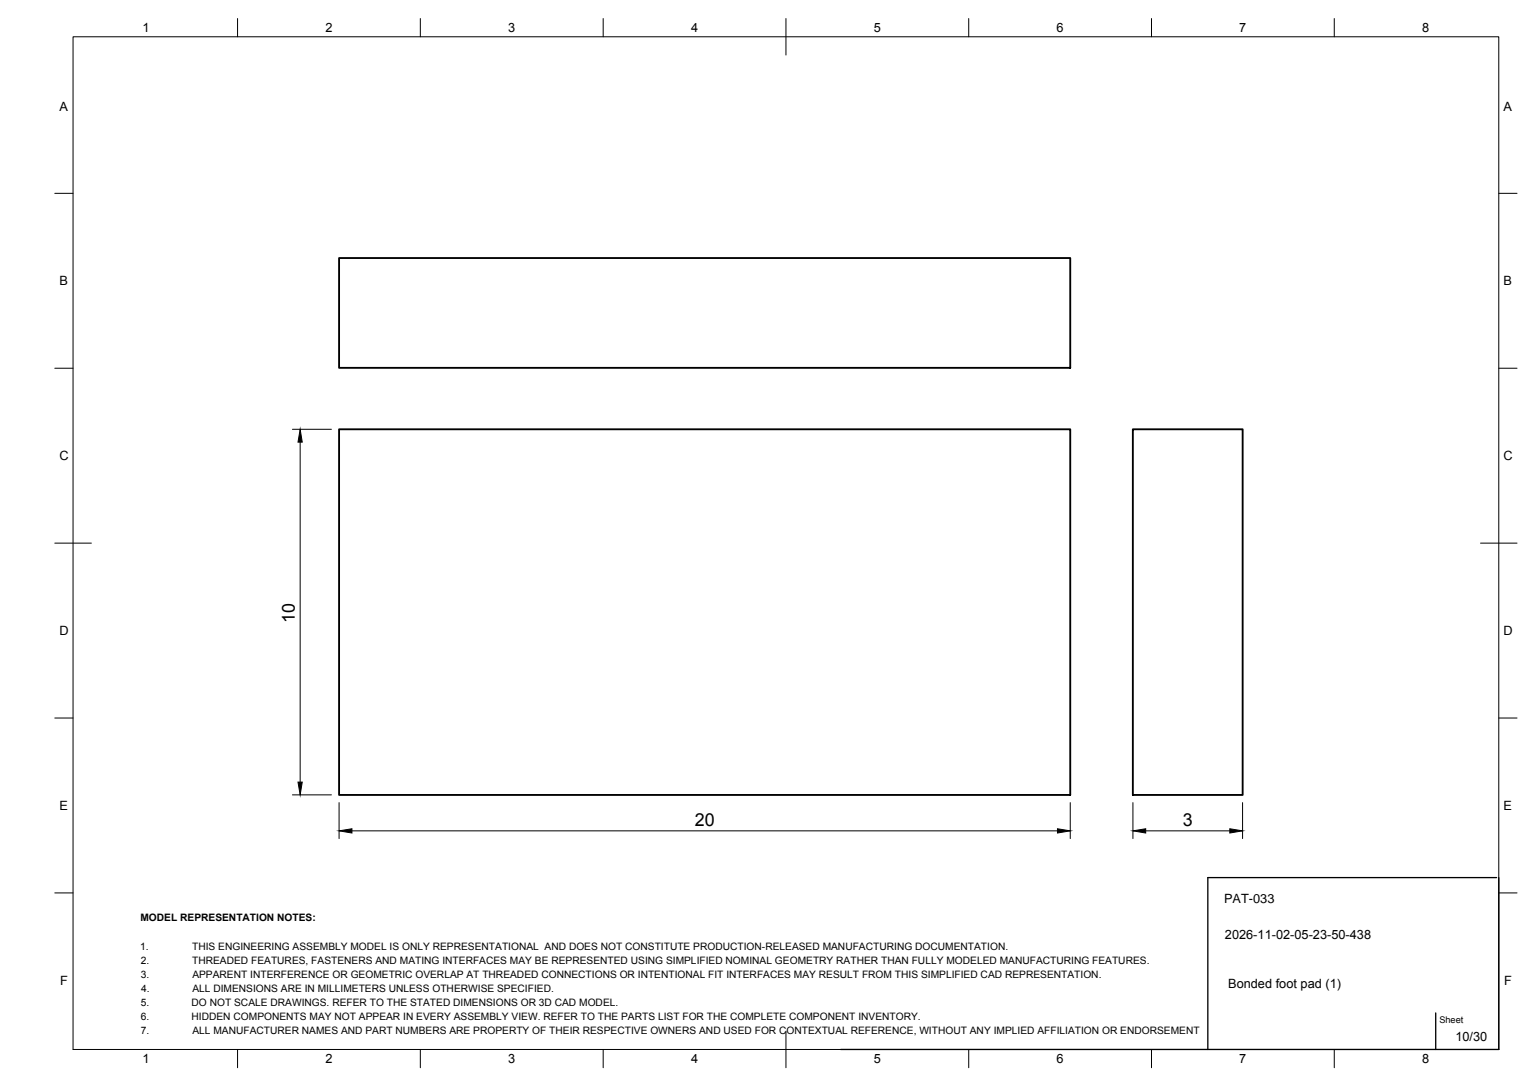
ISO-10303-21;
HEADER;
/* Generated by software containing ST-Developer
 * from STEP Tools, Inc. (www.steptools.com) 
 */

FILE_DESCRIPTION(
/* description */ ('Dual-rail gantry carriage'),
/* implementation_level */ '2;1');

FILE_NAME(
/* name */ 'Bonded foot pad (1).step',
/* time_stamp */ '2026-10-27T10:49:15-07:00',
/* author */ (''),
/* organization */ (''),
/* preprocessor_version */ 'ST-DEVELOPER v20.2',
/* originating_system */ 'Autodesk Translation Framework v15.17.0.0',
/* authorisation */ '');

FILE_SCHEMA (('AUTOMOTIVE_DESIGN { 1 0 10303 214 3 1 1 }'));
ENDSEC;

DATA;
#10=MECHANICAL_DESIGN_GEOMETRIC_PRESENTATION_REPRESENTATION('',(#590),#12804);
#528=SHAPE_REPRESENTATION_RELATIONSHIP('SRR','None',#13006,#559);
#559=ADVANCED_BREP_SHAPE_REPRESENTATION('',(#621),#12776);
#590=STYLED_ITEM('',(#13240),#621);
#621=MANIFOLD_SOLID_BREP('Body1',#7368);
#794=PLANE('',#7827);
#795=PLANE('',#7828);
#796=PLANE('',#7829);
#797=PLANE('',#7830);
#798=PLANE('',#7831);
#799=PLANE('',#7832);
#1094=FACE_OUTER_BOUND('',#1515,.T.);
#1095=FACE_OUTER_BOUND('',#1516,.T.);
#1096=FACE_OUTER_BOUND('',#1517,.T.);
#1097=FACE_OUTER_BOUND('',#1518,.T.);
#1098=FACE_OUTER_BOUND('',#1519,.T.);
#1099=FACE_OUTER_BOUND('',#1520,.T.);
#1515=EDGE_LOOP('',(#5283,#5284,#5285,#5286));
#1516=EDGE_LOOP('',(#5287,#5288,#5289,#5290));
#1517=EDGE_LOOP('',(#5291,#5292,#5293,#5294));
#1518=EDGE_LOOP('',(#5295,#5296,#5297,#5298));
#1519=EDGE_LOOP('',(#5299,#5300,#5301,#5302));
#1520=EDGE_LOOP('',(#5303,#5304,#5305,#5306));
#2024=LINE('',#10925,#2733);
#2025=LINE('',#10927,#2734);
#2026=LINE('',#10929,#2735);
#2027=LINE('',#10930,#2736);
#2028=LINE('',#10933,#2737);
#2029=LINE('',#10935,#2738);
#2030=LINE('',#10936,#2739);
#2031=LINE('',#10939,#2740);
#2032=LINE('',#10941,#2741);
#2033=LINE('',#10942,#2742);
#2034=LINE('',#10944,#2743);
#2035=LINE('',#10945,#2744);
#2733=VECTOR('',#8737,1.);
#2734=VECTOR('',#8738,1.);
#2735=VECTOR('',#8739,1.);
#2736=VECTOR('',#8740,1.);
#2737=VECTOR('',#8743,1.);
#2738=VECTOR('',#8744,1.);
#2739=VECTOR('',#8745,1.);
#2740=VECTOR('',#8748,1.);
#2741=VECTOR('',#8749,1.);
#2742=VECTOR('',#8750,1.);
#2743=VECTOR('',#8753,1.);
#2744=VECTOR('',#8754,1.);
#3638=VERTEX_POINT('',#10923);
#3639=VERTEX_POINT('',#10924);
#3640=VERTEX_POINT('',#10926);
#3641=VERTEX_POINT('',#10928);
#3642=VERTEX_POINT('',#10932);
#3643=VERTEX_POINT('',#10934);
#3644=VERTEX_POINT('',#10938);
#3645=VERTEX_POINT('',#10940);
#4264=EDGE_CURVE('',#3638,#3639,#2024,.T.);
#4265=EDGE_CURVE('',#3639,#3640,#2025,.T.);
#4266=EDGE_CURVE('',#3641,#3640,#2026,.T.);
#4267=EDGE_CURVE('',#3638,#3641,#2027,.T.);
#4268=EDGE_CURVE('',#3642,#3638,#2028,.T.);
#4269=EDGE_CURVE('',#3643,#3641,#2029,.T.);
#4270=EDGE_CURVE('',#3642,#3643,#2030,.T.);
#4271=EDGE_CURVE('',#3644,#3642,#2031,.T.);
#4272=EDGE_CURVE('',#3645,#3643,#2032,.T.);
#4273=EDGE_CURVE('',#3644,#3645,#2033,.T.);
#4274=EDGE_CURVE('',#3639,#3644,#2034,.T.);
#4275=EDGE_CURVE('',#3640,#3645,#2035,.T.);
#5283=ORIENTED_EDGE('',*,*,#4264,.T.);
#5284=ORIENTED_EDGE('',*,*,#4265,.T.);
#5285=ORIENTED_EDGE('',*,*,#4266,.F.);
#5286=ORIENTED_EDGE('',*,*,#4267,.F.);
#5287=ORIENTED_EDGE('',*,*,#4268,.T.);
#5288=ORIENTED_EDGE('',*,*,#4267,.T.);
#5289=ORIENTED_EDGE('',*,*,#4269,.F.);
#5290=ORIENTED_EDGE('',*,*,#4270,.F.);
#5291=ORIENTED_EDGE('',*,*,#4271,.T.);
#5292=ORIENTED_EDGE('',*,*,#4270,.T.);
#5293=ORIENTED_EDGE('',*,*,#4272,.F.);
#5294=ORIENTED_EDGE('',*,*,#4273,.F.);
#5295=ORIENTED_EDGE('',*,*,#4274,.T.);
#5296=ORIENTED_EDGE('',*,*,#4273,.T.);
#5297=ORIENTED_EDGE('',*,*,#4275,.F.);
#5298=ORIENTED_EDGE('',*,*,#4265,.F.);
#5299=ORIENTED_EDGE('',*,*,#4275,.T.);
#5300=ORIENTED_EDGE('',*,*,#4272,.T.);
#5301=ORIENTED_EDGE('',*,*,#4269,.T.);
#5302=ORIENTED_EDGE('',*,*,#4266,.T.);
#5303=ORIENTED_EDGE('',*,*,#4274,.F.);
#5304=ORIENTED_EDGE('',*,*,#4264,.F.);
#5305=ORIENTED_EDGE('',*,*,#4268,.F.);
#5306=ORIENTED_EDGE('',*,*,#4271,.F.);
#7020=ADVANCED_FACE('',(#1094),#794,.T.);
#7021=ADVANCED_FACE('',(#1095),#795,.T.);
#7022=ADVANCED_FACE('',(#1096),#796,.T.);
#7023=ADVANCED_FACE('',(#1097),#797,.T.);
#7024=ADVANCED_FACE('',(#1098),#798,.T.);
#7025=ADVANCED_FACE('',(#1099),#799,.F.);
#7368=CLOSED_SHELL('',(#7020,#7021,#7022,#7023,#7024,#7025));
#7826=AXIS2_PLACEMENT_3D('',#10921,#8733,#8734);
#7827=AXIS2_PLACEMENT_3D('',#10922,#8735,#8736);
#7828=AXIS2_PLACEMENT_3D('',#10931,#8741,#8742);
#7829=AXIS2_PLACEMENT_3D('',#10937,#8746,#8747);
#7830=AXIS2_PLACEMENT_3D('',#10943,#8751,#8752);
#7831=AXIS2_PLACEMENT_3D('',#10946,#8755,#8756);
#7832=AXIS2_PLACEMENT_3D('',#10947,#8757,#8758);
#8733=DIRECTION('axis',(0.,0.,1.));
#8734=DIRECTION('refdir',(1.,0.,0.));
#8735=DIRECTION('center_axis',(0.,1.,0.));
#8736=DIRECTION('ref_axis',(-1.,0.,0.));
#8737=DIRECTION('',(-1.,0.,0.));
#8738=DIRECTION('',(0.,0.,1.));
#8739=DIRECTION('',(-1.,0.,0.));
#8740=DIRECTION('',(0.,0.,1.));
#8741=DIRECTION('center_axis',(1.,0.,0.));
#8742=DIRECTION('ref_axis',(0.,1.,0.));
#8743=DIRECTION('',(0.,1.,0.));
#8744=DIRECTION('',(0.,1.,0.));
#8745=DIRECTION('',(0.,0.,1.));
#8746=DIRECTION('center_axis',(0.,-1.,0.));
#8747=DIRECTION('ref_axis',(1.,0.,0.));
#8748=DIRECTION('',(1.,0.,0.));
#8749=DIRECTION('',(1.,0.,0.));
#8750=DIRECTION('',(0.,0.,1.));
#8751=DIRECTION('center_axis',(-1.,0.,0.));
#8752=DIRECTION('ref_axis',(0.,-1.,0.));
#8753=DIRECTION('',(0.,-1.,0.));
#8754=DIRECTION('',(0.,-1.,0.));
#8755=DIRECTION('center_axis',(0.,0.,1.));
#8756=DIRECTION('ref_axis',(1.,0.,0.));
#8757=DIRECTION('center_axis',(0.,0.,1.));
#8758=DIRECTION('ref_axis',(1.,0.,0.));
#10921=CARTESIAN_POINT('',(0.,0.,0.));
#10922=CARTESIAN_POINT('Origin',(2.,12.5,-1.1));
#10923=CARTESIAN_POINT('',(2.,12.5,-1.1));
#10924=CARTESIAN_POINT('',(0.,12.5,-1.1));
#10925=CARTESIAN_POINT('',(2.,12.5,-1.1));
#10926=CARTESIAN_POINT('',(0.,12.5,-0.8));
#10927=CARTESIAN_POINT('',(0.,12.5,-1.1));
#10928=CARTESIAN_POINT('',(2.,12.5,-0.8));
#10929=CARTESIAN_POINT('',(2.,12.5,-0.8));
#10930=CARTESIAN_POINT('',(2.,12.5,-1.1));
#10931=CARTESIAN_POINT('Origin',(2.,11.5,-1.1));
#10932=CARTESIAN_POINT('',(2.,11.5,-1.1));
#10933=CARTESIAN_POINT('',(2.,11.5,-1.1));
#10934=CARTESIAN_POINT('',(2.,11.5,-0.8));
#10935=CARTESIAN_POINT('',(2.,11.5,-0.8));
#10936=CARTESIAN_POINT('',(2.,11.5,-1.1));
#10937=CARTESIAN_POINT('Origin',(0.,11.5,-1.1));
#10938=CARTESIAN_POINT('',(0.,11.5,-1.1));
#10939=CARTESIAN_POINT('',(0.,11.5,-1.1));
#10940=CARTESIAN_POINT('',(0.,11.5,-0.8));
#10941=CARTESIAN_POINT('',(0.,11.5,-0.8));
#10942=CARTESIAN_POINT('',(0.,11.5,-1.1));
#10943=CARTESIAN_POINT('Origin',(0.,12.5,-1.1));
#10944=CARTESIAN_POINT('',(0.,12.5,-1.1));
#10945=CARTESIAN_POINT('',(0.,12.5,-0.8));
#10946=CARTESIAN_POINT('Origin',(1.,12.,-0.8));
#10947=CARTESIAN_POINT('Origin',(1.,12.,-1.1));
#12740=UNCERTAINTY_MEASURE_WITH_UNIT(LENGTH_MEASURE(0.001),#12805,
'DISTANCE_ACCURACY_VALUE',
'Maximum model space distance between geometric entities at asserted c
onnectivities');
#12768=UNCERTAINTY_MEASURE_WITH_UNIT(LENGTH_MEASURE(0.001),#12805,
'DISTANCE_ACCURACY_VALUE',
'Maximum model space distance between geometric entities at asserted c
onnectivities');
#12776=(
GEOMETRIC_REPRESENTATION_CONTEXT(3)
GLOBAL_UNCERTAINTY_ASSIGNED_CONTEXT((#12740))
GLOBAL_UNIT_ASSIGNED_CONTEXT((#12805,#12807,#12808))
REPRESENTATION_CONTEXT('','3D')
);
#12804=(
GEOMETRIC_REPRESENTATION_CONTEXT(3)
GLOBAL_UNCERTAINTY_ASSIGNED_CONTEXT((#12768))
GLOBAL_UNIT_ASSIGNED_CONTEXT((#12805,#12807,#12808))
REPRESENTATION_CONTEXT('','3D')
);
#12805=(
LENGTH_UNIT()
NAMED_UNIT(*)
SI_UNIT(.CENTI.,.METRE.)
);
#12807=(
NAMED_UNIT(*)
PLANE_ANGLE_UNIT()
SI_UNIT($,.RADIAN.)
);
#12808=(
NAMED_UNIT(*)
SI_UNIT($,.STERADIAN.)
SOLID_ANGLE_UNIT()
);
#12816=SHAPE_DEFINITION_REPRESENTATION(#12851,#13006);
#12851=PRODUCT_DEFINITION_SHAPE('',$,#13042);
#13006=SHAPE_REPRESENTATION('',(#7826),#12776);
#13034=PRODUCT_DEFINITION_CONTEXT('part definition',#13141,'design');
#13042=PRODUCT_DEFINITION('Bonded foot pad (1)','Bonded foot pad (1)',#13077,
#13034);
#13077=PRODUCT_DEFINITION_FORMATION('',$,#13150);
#13141=APPLICATION_CONTEXT(
'Core Data for Automotive Mechanical Design Process');
#13142=PRODUCT_CONTEXT('part definition',#13141,'mechanical');
#13150=PRODUCT('Bonded foot pad (1)','Bonded foot pad (1)',
'Bonded foot pad (1)',(#13142));
#13234=COLOUR_RGB('Sky Blue',0.24,0.69,0.87);
#13235=FILL_AREA_STYLE_COLOUR('',#13234);
#13236=FILL_AREA_STYLE('',(#13235));
#13237=SURFACE_STYLE_FILL_AREA(#13236);
#13238=SURFACE_SIDE_STYLE('',(#13237));
#13239=SURFACE_STYLE_USAGE(.BOTH.,#13238);
#13240=PRESENTATION_STYLE_ASSIGNMENT((#13239));
ENDSEC;
END-ISO-10303-21;
